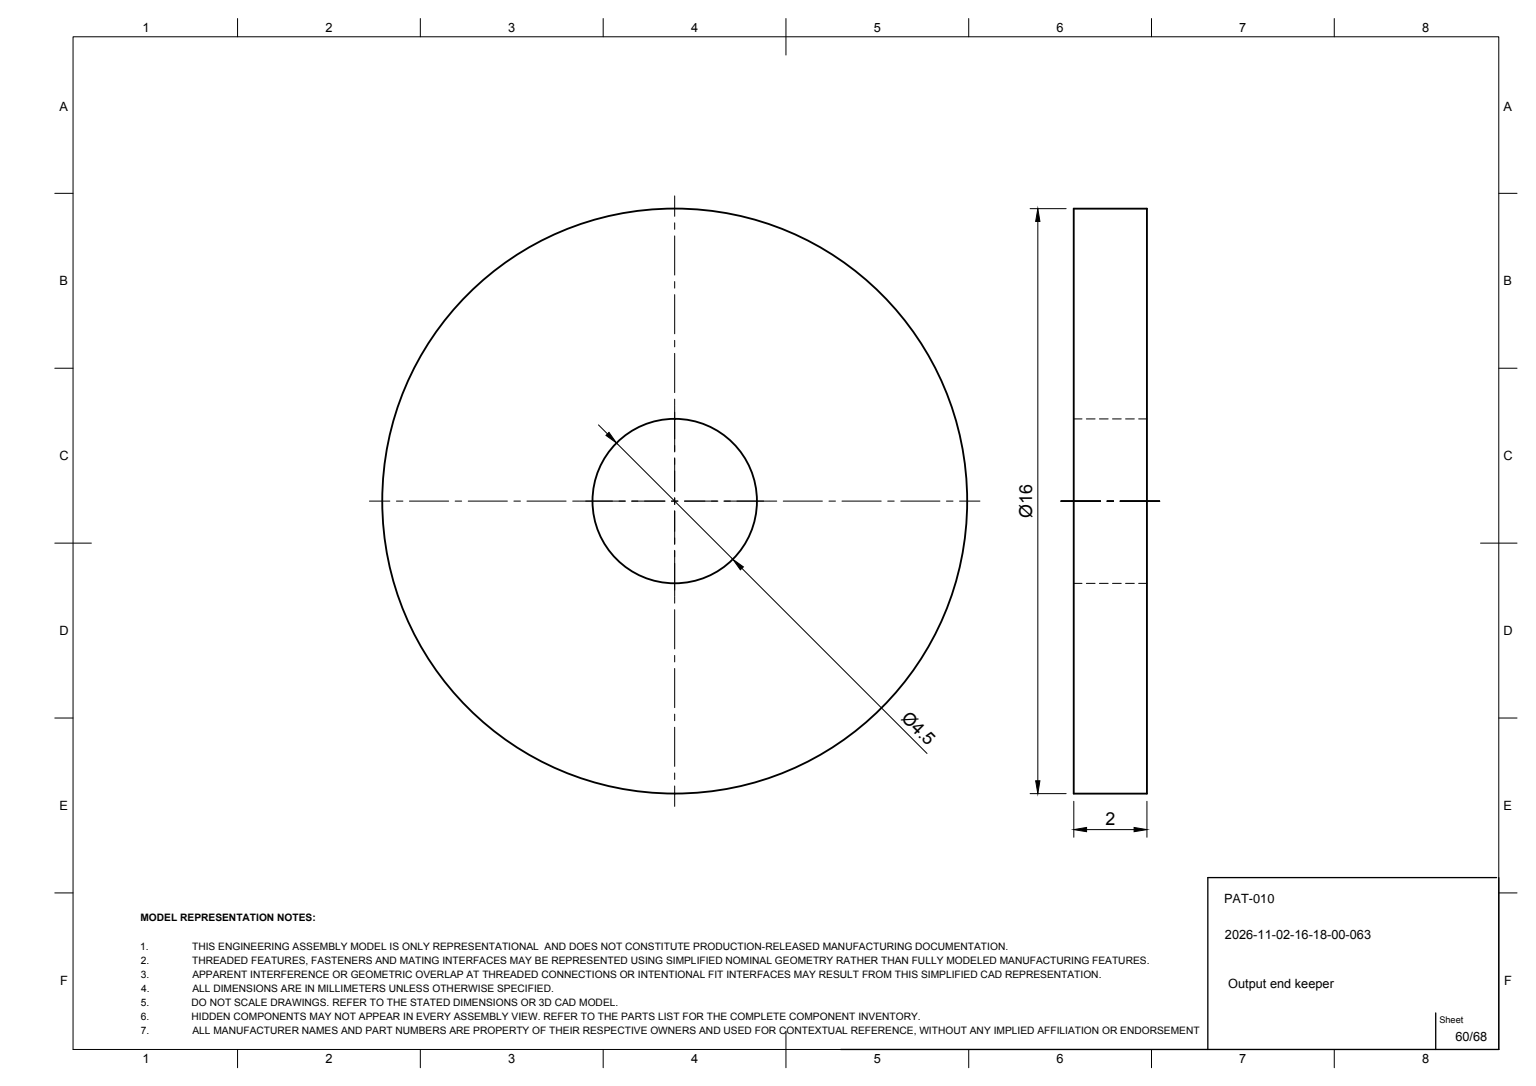
ISO-10303-21;
HEADER;
/* Generated by software containing ST-Developer
 * from STEP Tools, Inc. (www.steptools.com) 
 */

FILE_DESCRIPTION(
/* description */ ('Belt conveyor head drive unit'),
/* implementation_level */ '2;1');

FILE_NAME(
/* name */ 'Output end keeper.step',
/* time_stamp */ '2026-10-28T03:26:19-07:00',
/* author */ (''),
/* organization */ (''),
/* preprocessor_version */ 'ST-DEVELOPER v20.2',
/* originating_system */ 'Autodesk Translation Framework v15.17.0.0',
/* authorisation */ '');

FILE_SCHEMA (('AUTOMOTIVE_DESIGN { 1 0 10303 214 3 1 1 }'));
ENDSEC;

DATA;
#10=MECHANICAL_DESIGN_GEOMETRIC_PRESENTATION_REPRESENTATION('',(#921),#27069);
#767=SHAPE_REPRESENTATION_RELATIONSHIP('SRR','None',#27416,#836);
#836=ADVANCED_BREP_SHAPE_REPRESENTATION('',(#1002),#27058);
#921=STYLED_ITEM('',(#27811),#1002);
#1002=MANIFOLD_SOLID_BREP('Body1',#13790);
#1240=FACE_BOUND('',#3298,.T.);
#1241=FACE_BOUND('',#3300,.T.);
#1584=PLANE('',#15927);
#1585=PLANE('',#15928);
#2267=FACE_OUTER_BOUND('',#3295,.T.);
#2268=FACE_OUTER_BOUND('',#3296,.T.);
#2269=FACE_OUTER_BOUND('',#3297,.T.);
#2270=FACE_OUTER_BOUND('',#3299,.T.);
#3295=EDGE_LOOP('',(#11682,#11683,#11684,#11685));
#3296=EDGE_LOOP('',(#11686,#11687,#11688,#11689));
#3297=EDGE_LOOP('',(#11690));
#3298=EDGE_LOOP('',(#11691));
#3299=EDGE_LOOP('',(#11692));
#3300=EDGE_LOOP('',(#11693));
#4127=LINE('',#25402,#4919);
#4128=LINE('',#25408,#4920);
#4919=VECTOR('',#19785,0.225);
#4920=VECTOR('',#19792,0.8);
#5729=CIRCLE('',#15922,0.225);
#5730=CIRCLE('',#15923,0.225);
#5731=CIRCLE('',#15925,0.8);
#5732=CIRCLE('',#15926,0.8);
#6885=VERTEX_POINT('',#25399);
#6886=VERTEX_POINT('',#25401);
#6887=VERTEX_POINT('',#25405);
#6888=VERTEX_POINT('',#25407);
#8533=EDGE_CURVE('',#6885,#6885,#5729,.T.);
#8534=EDGE_CURVE('',#6885,#6886,#4127,.T.);
#8535=EDGE_CURVE('',#6886,#6886,#5730,.T.);
#8536=EDGE_CURVE('',#6887,#6887,#5731,.T.);
#8537=EDGE_CURVE('',#6887,#6888,#4128,.T.);
#8538=EDGE_CURVE('',#6888,#6888,#5732,.T.);
#11682=ORIENTED_EDGE('',*,*,#8533,.F.);
#11683=ORIENTED_EDGE('',*,*,#8534,.T.);
#11684=ORIENTED_EDGE('',*,*,#8535,.T.);
#11685=ORIENTED_EDGE('',*,*,#8534,.F.);
#11686=ORIENTED_EDGE('',*,*,#8536,.F.);
#11687=ORIENTED_EDGE('',*,*,#8537,.T.);
#11688=ORIENTED_EDGE('',*,*,#8538,.T.);
#11689=ORIENTED_EDGE('',*,*,#8537,.F.);
#11690=ORIENTED_EDGE('',*,*,#8536,.T.);
#11691=ORIENTED_EDGE('',*,*,#8533,.T.);
#11692=ORIENTED_EDGE('',*,*,#8538,.F.);
#11693=ORIENTED_EDGE('',*,*,#8535,.F.);
#12801=CYLINDRICAL_SURFACE('',#15921,0.225);
#12802=CYLINDRICAL_SURFACE('',#15924,0.8);
#13546=ADVANCED_FACE('',(#2267),#12801,.F.);
#13547=ADVANCED_FACE('',(#2268),#12802,.T.);
#13548=ADVANCED_FACE('',(#2269,#1240),#1584,.T.);
#13549=ADVANCED_FACE('',(#2270,#1241),#1585,.F.);
#13790=CLOSED_SHELL('',(#13546,#13547,#13548,#13549));
#15920=AXIS2_PLACEMENT_3D('',#25397,#19779,#19780);
#15921=AXIS2_PLACEMENT_3D('',#25398,#19781,#19782);
#15922=AXIS2_PLACEMENT_3D('',#25400,#19783,#19784);
#15923=AXIS2_PLACEMENT_3D('',#25403,#19786,#19787);
#15924=AXIS2_PLACEMENT_3D('',#25404,#19788,#19789);
#15925=AXIS2_PLACEMENT_3D('',#25406,#19790,#19791);
#15926=AXIS2_PLACEMENT_3D('',#25409,#19793,#19794);
#15927=AXIS2_PLACEMENT_3D('',#25410,#19795,#19796);
#15928=AXIS2_PLACEMENT_3D('',#25411,#19797,#19798);
#19779=DIRECTION('axis',(0.,0.,1.));
#19780=DIRECTION('refdir',(1.,0.,0.));
#19781=DIRECTION('center_axis',(0.,1.,0.));
#19782=DIRECTION('ref_axis',(1.,0.,0.));
#19783=DIRECTION('center_axis',(0.,-1.,0.));
#19784=DIRECTION('ref_axis',(1.,0.,0.));
#19785=DIRECTION('',(0.,-1.,0.));
#19786=DIRECTION('center_axis',(0.,-1.,0.));
#19787=DIRECTION('ref_axis',(1.,0.,0.));
#19788=DIRECTION('center_axis',(0.,1.,0.));
#19789=DIRECTION('ref_axis',(1.,0.,0.));
#19790=DIRECTION('center_axis',(0.,1.,0.));
#19791=DIRECTION('ref_axis',(1.,0.,0.));
#19792=DIRECTION('',(0.,-1.,0.));
#19793=DIRECTION('center_axis',(0.,1.,0.));
#19794=DIRECTION('ref_axis',(1.,0.,0.));
#19795=DIRECTION('center_axis',(0.,1.,0.));
#19796=DIRECTION('ref_axis',(1.,0.,0.));
#19797=DIRECTION('center_axis',(0.,1.,0.));
#19798=DIRECTION('ref_axis',(1.,0.,0.));
#25397=CARTESIAN_POINT('',(0.,0.,0.));
#25398=CARTESIAN_POINT('Origin',(6.97091003018116,-5.2,7.));
#25399=CARTESIAN_POINT('',(6.74591003018116,-5.,7.));
#25400=CARTESIAN_POINT('Origin',(6.97091003018116,-5.,7.));
#25401=CARTESIAN_POINT('',(6.74591003018116,-5.2,7.));
#25402=CARTESIAN_POINT('',(6.74591003018116,-5.2,7.));
#25403=CARTESIAN_POINT('Origin',(6.97091003018116,-5.2,7.));
#25404=CARTESIAN_POINT('Origin',(6.97091003018116,-5.2,7.));
#25405=CARTESIAN_POINT('',(6.17091003018116,-5.,7.));
#25406=CARTESIAN_POINT('Origin',(6.97091003018116,-5.,7.));
#25407=CARTESIAN_POINT('',(6.17091003018116,-5.2,7.));
#25408=CARTESIAN_POINT('',(6.17091003018116,-5.2,7.));
#25409=CARTESIAN_POINT('Origin',(6.97091003018116,-5.2,7.));
#25410=CARTESIAN_POINT('Origin',(6.97091003018116,-5.,7.));
#25411=CARTESIAN_POINT('Origin',(6.97091003018116,-5.2,7.));
#26981=UNCERTAINTY_MEASURE_WITH_UNIT(LENGTH_MEASURE(0.001),#27070,
'DISTANCE_ACCURACY_VALUE',
'Maximum model space distance between geometric entities at asserted c
onnectivities');
#26992=UNCERTAINTY_MEASURE_WITH_UNIT(LENGTH_MEASURE(0.001),#27070,
'DISTANCE_ACCURACY_VALUE',
'Maximum model space distance between geometric entities at asserted c
onnectivities');
#27058=(
GEOMETRIC_REPRESENTATION_CONTEXT(3)
GLOBAL_UNCERTAINTY_ASSIGNED_CONTEXT((#26981))
GLOBAL_UNIT_ASSIGNED_CONTEXT((#27070,#27072,#27073))
REPRESENTATION_CONTEXT('','3D')
);
#27069=(
GEOMETRIC_REPRESENTATION_CONTEXT(3)
GLOBAL_UNCERTAINTY_ASSIGNED_CONTEXT((#26992))
GLOBAL_UNIT_ASSIGNED_CONTEXT((#27070,#27072,#27073))
REPRESENTATION_CONTEXT('','3D')
);
#27070=(
LENGTH_UNIT()
NAMED_UNIT(*)
SI_UNIT(.CENTI.,.METRE.)
);
#27072=(
NAMED_UNIT(*)
PLANE_ANGLE_UNIT()
SI_UNIT($,.RADIAN.)
);
#27073=(
NAMED_UNIT(*)
SI_UNIT($,.STERADIAN.)
SOLID_ANGLE_UNIT()
);
#27139=SHAPE_DEFINITION_REPRESENTATION(#27227,#27416);
#27227=PRODUCT_DEFINITION_SHAPE('',$,#27493);
#27416=SHAPE_REPRESENTATION('',(#15920),#27058);
#27427=PRODUCT_DEFINITION_CONTEXT('part definition',#27657,'design');
#27493=PRODUCT_DEFINITION('Output end keeper','Output end keeper',#27569,
#27427);
#27569=PRODUCT_DEFINITION_FORMATION('',$,#27724);
#27657=APPLICATION_CONTEXT(
'Core Data for Automotive Mechanical Design Process');
#27658=PRODUCT_CONTEXT('part definition',#27657,'mechanical');
#27724=PRODUCT('Output end keeper','Output end keeper',
'Output end keeper',(#27658));
#27805=COLOUR_RGB('Off White',0.89,0.88,0.83);
#27806=FILL_AREA_STYLE_COLOUR('',#27805);
#27807=FILL_AREA_STYLE('',(#27806));
#27808=SURFACE_STYLE_FILL_AREA(#27807);
#27809=SURFACE_SIDE_STYLE('',(#27808));
#27810=SURFACE_STYLE_USAGE(.BOTH.,#27809);
#27811=PRESENTATION_STYLE_ASSIGNMENT((#27810));
ENDSEC;
END-ISO-10303-21;
